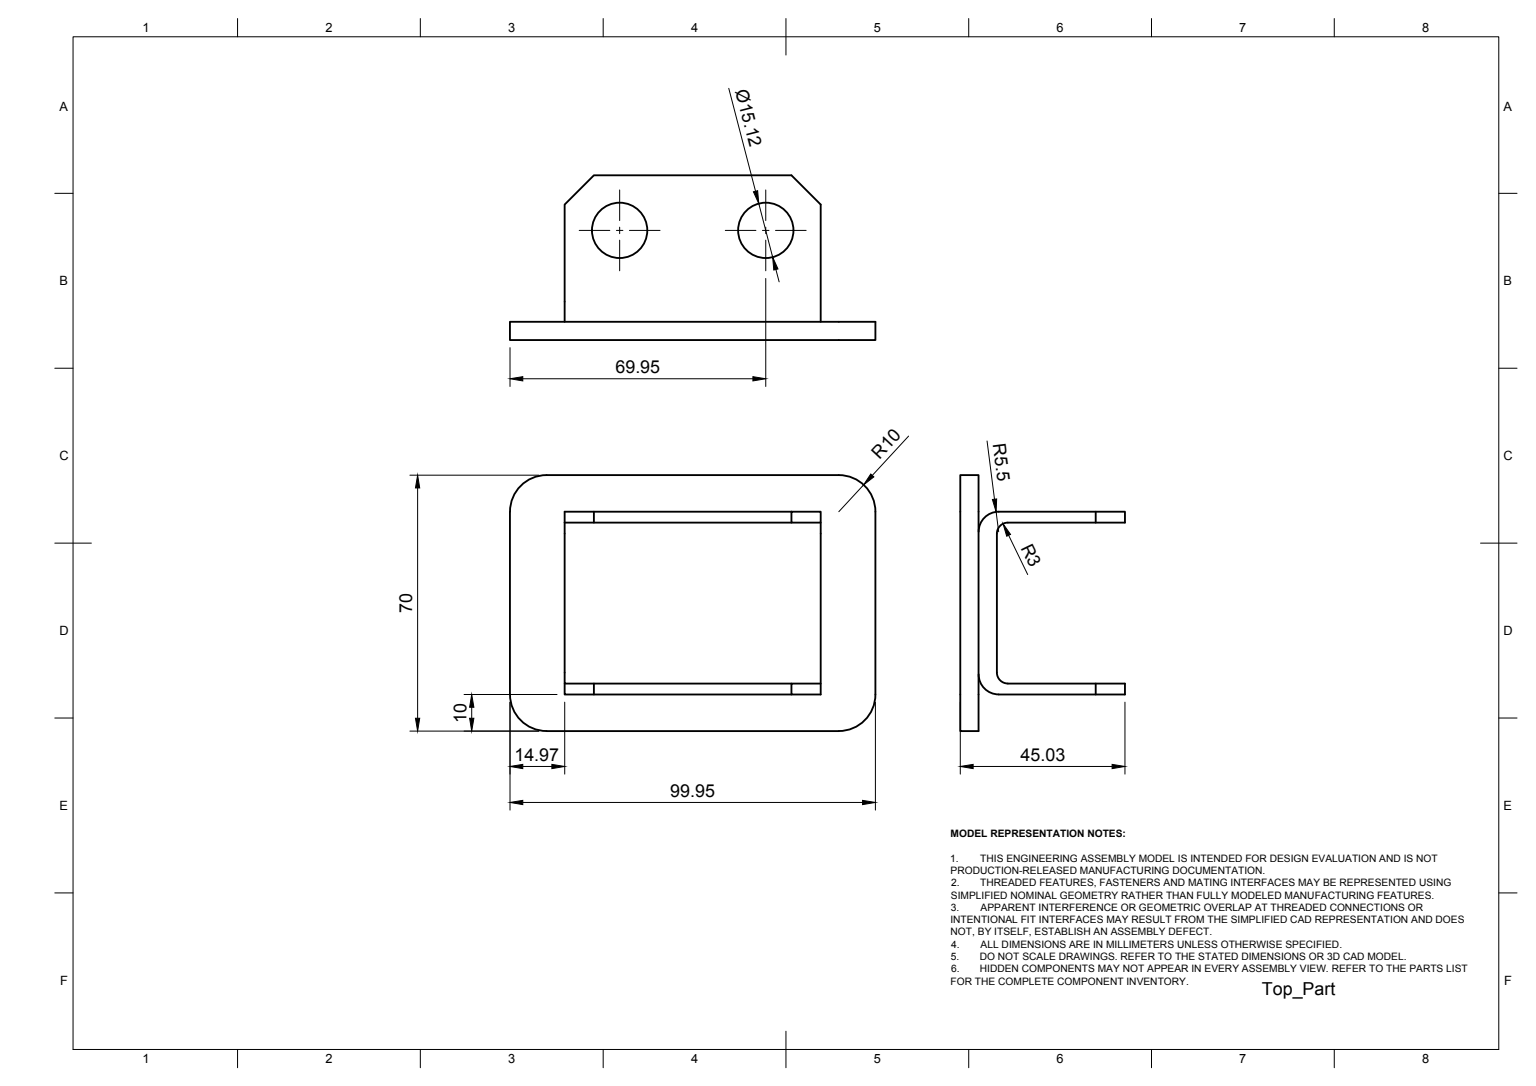
ISO-10303-21;
HEADER;
/* Generated by software containing ST-Developer
 * from STEP Tools, Inc. (www.steptools.com) 
 */

FILE_DESCRIPTION(
/* description */ (''),
/* implementation_level */ '2;1');

FILE_NAME(
/* name */ 'Top_Part.step',
/* time_stamp */ '2026-10-06T13:41:14-07:00',
/* author */ (''),
/* organization */ (''),
/* preprocessor_version */ 'ST-DEVELOPER v20.2',
/* originating_system */ 'Autodesk Translation Framework v15.15.0.0',
/* authorisation */ '');

FILE_SCHEMA (('AUTOMOTIVE_DESIGN { 1 0 10303 214 3 1 1 }'));
ENDSEC;

DATA;
#10=MECHANICAL_DESIGN_GEOMETRIC_PRESENTATION_REPRESENTATION('',(#1966),#279266);
#1948=SHAPE_REPRESENTATION_RELATIONSHIP('SRR','None',#279307,#1957);
#1957=ADVANCED_BREP_SHAPE_REPRESENTATION('',(#1975),#279263);
#1966=STYLED_ITEM('',(#279355),#1975);
#1975=MANIFOLD_SOLID_BREP('Body1',#14944);
#2008=FACE_BOUND('',#3013,.T.);
#2009=FACE_BOUND('',#3014,.T.);
#2010=FACE_BOUND('',#3017,.T.);
#2011=FACE_BOUND('',#3018,.T.);
#2012=FACE_BOUND('',#3030,.T.);
#2013=FACE_BOUND('',#3035,.T.);
#2014=FACE_BOUND('',#3036,.T.);
#2015=FACE_BOUND('',#3039,.T.);
#2016=FACE_BOUND('',#3040,.T.);
#2081=PLANE('',#15559);
#2082=PLANE('',#15563);
#2083=PLANE('',#15567);
#2084=PLANE('',#15572);
#2085=PLANE('',#15575);
#2086=PLANE('',#15576);
#2087=PLANE('',#15580);
#2088=PLANE('',#15581);
#2089=PLANE('',#15587);
#2090=PLANE('',#15591);
#2091=PLANE('',#15592);
#2092=PLANE('',#15593);
#2093=PLANE('',#15594);
#2094=PLANE('',#15597);
#2095=PLANE('',#15601);
#2096=PLANE('',#15603);
#2097=PLANE('',#15605);
#2098=PLANE('',#15606);
#2099=PLANE('',#15607);
#2506=FACE_OUTER_BOUND('',#3006,.T.);
#2507=FACE_OUTER_BOUND('',#3007,.T.);
#2508=FACE_OUTER_BOUND('',#3008,.T.);
#2509=FACE_OUTER_BOUND('',#3009,.T.);
#2510=FACE_OUTER_BOUND('',#3010,.T.);
#2511=FACE_OUTER_BOUND('',#3011,.T.);
#2512=FACE_OUTER_BOUND('',#3012,.T.);
#2513=FACE_OUTER_BOUND('',#3015,.T.);
#2514=FACE_OUTER_BOUND('',#3016,.T.);
#2515=FACE_OUTER_BOUND('',#3019,.T.);
#2516=FACE_OUTER_BOUND('',#3020,.T.);
#2517=FACE_OUTER_BOUND('',#3021,.T.);
#2518=FACE_OUTER_BOUND('',#3022,.T.);
#2519=FACE_OUTER_BOUND('',#3023,.T.);
#2520=FACE_OUTER_BOUND('',#3024,.T.);
#2521=FACE_OUTER_BOUND('',#3025,.T.);
#2522=FACE_OUTER_BOUND('',#3026,.T.);
#2523=FACE_OUTER_BOUND('',#3027,.T.);
#2524=FACE_OUTER_BOUND('',#3028,.T.);
#2525=FACE_OUTER_BOUND('',#3029,.T.);
#2526=FACE_OUTER_BOUND('',#3031,.T.);
#2527=FACE_OUTER_BOUND('',#3032,.T.);
#2528=FACE_OUTER_BOUND('',#3033,.T.);
#2529=FACE_OUTER_BOUND('',#3034,.T.);
#2530=FACE_OUTER_BOUND('',#3037,.T.);
#2531=FACE_OUTER_BOUND('',#3038,.T.);
#2532=FACE_OUTER_BOUND('',#3041,.T.);
#2533=FACE_OUTER_BOUND('',#3042,.T.);
#2534=FACE_OUTER_BOUND('',#3043,.T.);
#2535=FACE_OUTER_BOUND('',#3044,.T.);
#2536=FACE_OUTER_BOUND('',#3045,.T.);
#3006=EDGE_LOOP('',(#13550,#13551,#13552,#13553));
#3007=EDGE_LOOP('',(#13554,#13555,#13556,#13557));
#3008=EDGE_LOOP('',(#13558,#13559,#13560,#13561));
#3009=EDGE_LOOP('',(#13562,#13563,#13564,#13565));
#3010=EDGE_LOOP('',(#13566,#13567,#13568,#13569));
#3011=EDGE_LOOP('',(#13570,#13571,#13572,#13573));
#3012=EDGE_LOOP('',(#13574,#13575,#13576,#13577,#13578,#13579));
#3013=EDGE_LOOP('',(#13580));
#3014=EDGE_LOOP('',(#13581));
#3015=EDGE_LOOP('',(#13582,#13583,#13584,#13585));
#3016=EDGE_LOOP('',(#13586,#13587,#13588,#13589,#13590,#13591));
#3017=EDGE_LOOP('',(#13592));
#3018=EDGE_LOOP('',(#13593));
#3019=EDGE_LOOP('',(#13594,#13595,#13596,#13597));
#3020=EDGE_LOOP('',(#13598,#13599,#13600,#13601));
#3021=EDGE_LOOP('',(#13602,#13603,#13604,#13605));
#3022=EDGE_LOOP('',(#13606,#13607,#13608,#13609));
#3023=EDGE_LOOP('',(#13610,#13611,#13612,#13613));
#3024=EDGE_LOOP('',(#13614,#13615,#13616,#13617,#13618,#13619,#13620,#13621,
#13622,#13623,#13624,#13625));
#3025=EDGE_LOOP('',(#13626,#13627,#13628,#13629));
#3026=EDGE_LOOP('',(#13630,#13631,#13632,#13633));
#3027=EDGE_LOOP('',(#13634,#13635,#13636,#13637));
#3028=EDGE_LOOP('',(#13638,#13639,#13640,#13641));
#3029=EDGE_LOOP('',(#13642,#13643,#13644,#13645,#13646,#13647,#13648,#13649));
#3030=EDGE_LOOP('',(#13650,#13651,#13652,#13653));
#3031=EDGE_LOOP('',(#13654,#13655,#13656,#13657));
#3032=EDGE_LOOP('',(#13658,#13659,#13660,#13661,#13662,#13663,#13664,#13665));
#3033=EDGE_LOOP('',(#13666,#13667,#13668,#13669));
#3034=EDGE_LOOP('',(#13670,#13671,#13672,#13673,#13674,#13675));
#3035=EDGE_LOOP('',(#13676));
#3036=EDGE_LOOP('',(#13677));
#3037=EDGE_LOOP('',(#13678,#13679,#13680,#13681));
#3038=EDGE_LOOP('',(#13682,#13683,#13684,#13685,#13686,#13687));
#3039=EDGE_LOOP('',(#13688));
#3040=EDGE_LOOP('',(#13689));
#3041=EDGE_LOOP('',(#13690,#13691,#13692,#13693,#13694,#13695,#13696,#13697,
#13698,#13699,#13700,#13701));
#3042=EDGE_LOOP('',(#13702,#13703,#13704,#13705));
#3043=EDGE_LOOP('',(#13706,#13707,#13708,#13709));
#3044=EDGE_LOOP('',(#13710,#13711,#13712,#13713));
#3045=EDGE_LOOP('',(#13714,#13715,#13716,#13717));
#3525=LINE('',#240639,#4053);
#3526=LINE('',#240642,#4054);
#3527=LINE('',#240647,#4055);
#3528=LINE('',#240652,#4056);
#3529=LINE('',#240654,#4057);
#3530=LINE('',#240656,#4058);
#3531=LINE('',#240657,#4059);
#3532=LINE('',#240663,#4060);
#3533=LINE('',#240666,#4061);
#3534=LINE('',#240668,#4062);
#3535=LINE('',#240669,#4063);
#3536=LINE('',#240673,#4064);
#3537=LINE('',#240677,#4065);
#3538=LINE('',#240680,#4066);
#3539=LINE('',#240682,#4067);
#3540=LINE('',#240684,#4068);
#3541=LINE('',#240685,#4069);
#3542=LINE('',#240693,#4070);
#3543=LINE('',#240696,#4071);
#3544=LINE('',#240699,#4072);
#3545=LINE('',#240701,#4073);
#3546=LINE('',#240702,#4074);
#3547=LINE('',#240703,#4075);
#3548=LINE('',#240707,#4076);
#3549=LINE('',#240709,#4077);
#3550=LINE('',#240711,#4078);
#3551=LINE('',#240717,#4079);
#3552=LINE('',#240720,#4080);
#3553=LINE('',#240722,#4081);
#3554=LINE('',#240723,#4082);
#3555=LINE('',#240728,#4083);
#3556=LINE('',#240730,#4084);
#3557=LINE('',#240734,#4085);
#3558=LINE('',#240736,#4086);
#3559=LINE('',#240737,#4087);
#3560=LINE('',#240742,#4088);
#3561=LINE('',#240746,#4089);
#3562=LINE('',#240748,#4090);
#3563=LINE('',#240749,#4091);
#3564=LINE('',#240755,#4092);
#3565=LINE('',#240758,#4093);
#3566=LINE('',#240760,#4094);
#3567=LINE('',#240761,#4095);
#3568=LINE('',#240763,#4096);
#3569=LINE('',#240765,#4097);
#3570=LINE('',#240766,#4098);
#3571=LINE('',#240768,#4099);
#3572=LINE('',#240772,#4100);
#3573=LINE('',#240774,#4101);
#3574=LINE('',#240778,#4102);
#3575=LINE('',#240780,#4103);
#3576=LINE('',#240781,#4104);
#3577=LINE('',#240787,#4105);
#3578=LINE('',#240790,#4106);
#3579=LINE('',#240792,#4107);
#3580=LINE('',#240793,#4108);
#3581=LINE('',#240797,#4109);
#3582=LINE('',#240798,#4110);
#3583=LINE('',#240800,#4111);
#3584=LINE('',#240802,#4112);
#4053=VECTOR('',#17119,10.);
#4054=VECTOR('',#17122,10.);
#4055=VECTOR('',#17127,7.55784864301595);
#4056=VECTOR('',#17132,10.);
#4057=VECTOR('',#17133,10.);
#4058=VECTOR('',#17134,9.99999999999999);
#4059=VECTOR('',#17135,10.);
#4060=VECTOR('',#17140,10.);
#4061=VECTOR('',#17143,10.);
#4062=VECTOR('',#17146,10.);
#4063=VECTOR('',#17147,10.);
#4064=VECTOR('',#17150,10.);
#4065=VECTOR('',#17153,10.);
#4066=VECTOR('',#17158,10.);
#4067=VECTOR('',#17159,10.);
#4068=VECTOR('',#17160,10.);
#4069=VECTOR('',#17161,10.);
#4070=VECTOR('',#17168,10.);
#4071=VECTOR('',#17171,10.);
#4072=VECTOR('',#17174,10.);
#4073=VECTOR('',#17175,9.99999999999999);
#4074=VECTOR('',#17176,10.);
#4075=VECTOR('',#17177,10.);
#4076=VECTOR('',#17182,7.55784864301595);
#4077=VECTOR('',#17185,10.);
#4078=VECTOR('',#17188,10.);
#4079=VECTOR('',#17193,10.);
#4080=VECTOR('',#17196,10.);
#4081=VECTOR('',#17199,10.);
#4082=VECTOR('',#17200,10.);
#4083=VECTOR('',#17205,10.);
#4084=VECTOR('',#17206,10.);
#4085=VECTOR('',#17209,10.);
#4086=VECTOR('',#17210,10.);
#4087=VECTOR('',#17211,10.);
#4088=VECTOR('',#17216,7.55784864301595);
#4089=VECTOR('',#17221,10.);
#4090=VECTOR('',#17222,10.);
#4091=VECTOR('',#17223,9.99999999999999);
#4092=VECTOR('',#17228,10.);
#4093=VECTOR('',#17231,10.);
#4094=VECTOR('',#17234,10.);
#4095=VECTOR('',#17235,10.);
#4096=VECTOR('',#17238,10.);
#4097=VECTOR('',#17239,10.);
#4098=VECTOR('',#17240,10.);
#4099=VECTOR('',#17243,10.);
#4100=VECTOR('',#17248,10.);
#4101=VECTOR('',#17249,10.);
#4102=VECTOR('',#17254,10.);
#4103=VECTOR('',#17255,10.);
#4104=VECTOR('',#17256,10.);
#4105=VECTOR('',#17263,10.);
#4106=VECTOR('',#17266,10.);
#4107=VECTOR('',#17267,9.99999999999999);
#4108=VECTOR('',#17268,10.);
#4109=VECTOR('',#17273,10.);
#4110=VECTOR('',#17274,10.);
#4111=VECTOR('',#17277,7.55784864301595);
#4112=VECTOR('',#17280,10.);
#4260=CIRCLE('',#15554,10.);
#4261=CIRCLE('',#15555,10.);
#4262=CIRCLE('',#15557,7.55784864301595);
#4263=CIRCLE('',#15558,7.55784864301595);
#4264=CIRCLE('',#15561,10.);
#4265=CIRCLE('',#15562,10.);
#4266=CIRCLE('',#15565,3.);
#4267=CIRCLE('',#15566,3.);
#4268=CIRCLE('',#15568,7.55784864301595);
#4269=CIRCLE('',#15570,5.5);
#4270=CIRCLE('',#15571,5.5);
#4271=CIRCLE('',#15573,7.55784864301595);
#4272=CIRCLE('',#15578,10.);
#4273=CIRCLE('',#15579,10.);
#4274=CIRCLE('',#15582,5.5);
#4275=CIRCLE('',#15583,3.);
#4276=CIRCLE('',#15585,7.55784864301595);
#4277=CIRCLE('',#15586,7.55784864301595);
#4278=CIRCLE('',#15589,10.);
#4279=CIRCLE('',#15590,10.);
#4280=CIRCLE('',#15596,3.);
#4281=CIRCLE('',#15598,7.55784864301595);
#4282=CIRCLE('',#15600,5.5);
#4283=CIRCLE('',#15602,7.55784864301595);
#6207=VERTEX_POINT('',#240635);
#6208=VERTEX_POINT('',#240636);
#6209=VERTEX_POINT('',#240638);
#6210=VERTEX_POINT('',#240640);
#6211=VERTEX_POINT('',#240644);
#6212=VERTEX_POINT('',#240646);
#6213=VERTEX_POINT('',#240650);
#6214=VERTEX_POINT('',#240651);
#6215=VERTEX_POINT('',#240653);
#6216=VERTEX_POINT('',#240655);
#6217=VERTEX_POINT('',#240659);
#6218=VERTEX_POINT('',#240660);
#6219=VERTEX_POINT('',#240662);
#6220=VERTEX_POINT('',#240664);
#6221=VERTEX_POINT('',#240671);
#6222=VERTEX_POINT('',#240672);
#6223=VERTEX_POINT('',#240674);
#6224=VERTEX_POINT('',#240676);
#6225=VERTEX_POINT('',#240681);
#6226=VERTEX_POINT('',#240683);
#6227=VERTEX_POINT('',#240686);
#6228=VERTEX_POINT('',#240689);
#6229=VERTEX_POINT('',#240690);
#6230=VERTEX_POINT('',#240692);
#6231=VERTEX_POINT('',#240694);
#6232=VERTEX_POINT('',#240698);
#6233=VERTEX_POINT('',#240700);
#6234=VERTEX_POINT('',#240704);
#6235=VERTEX_POINT('',#240713);
#6236=VERTEX_POINT('',#240714);
#6237=VERTEX_POINT('',#240716);
#6238=VERTEX_POINT('',#240718);
#6239=VERTEX_POINT('',#240725);
#6240=VERTEX_POINT('',#240726);
#6241=VERTEX_POINT('',#240729);
#6242=VERTEX_POINT('',#240731);
#6243=VERTEX_POINT('',#240733);
#6244=VERTEX_POINT('',#240735);
#6245=VERTEX_POINT('',#240739);
#6246=VERTEX_POINT('',#240741);
#6247=VERTEX_POINT('',#240745);
#6248=VERTEX_POINT('',#240747);
#6249=VERTEX_POINT('',#240751);
#6250=VERTEX_POINT('',#240752);
#6251=VERTEX_POINT('',#240754);
#6252=VERTEX_POINT('',#240756);
#6253=VERTEX_POINT('',#240764);
#6254=VERTEX_POINT('',#240771);
#6255=VERTEX_POINT('',#240773);
#6256=VERTEX_POINT('',#240777);
#6257=VERTEX_POINT('',#240779);
#6258=VERTEX_POINT('',#240782);
#6259=VERTEX_POINT('',#240785);
#6260=VERTEX_POINT('',#240789);
#6261=VERTEX_POINT('',#240791);
#6262=VERTEX_POINT('',#240794);
#8700=EDGE_CURVE('',#6207,#6208,#4260,.T.);
#8701=EDGE_CURVE('',#6209,#6207,#3525,.T.);
#8702=EDGE_CURVE('',#6210,#6209,#4261,.T.);
#8703=EDGE_CURVE('',#6208,#6210,#3526,.T.);
#8704=EDGE_CURVE('',#6211,#6211,#4262,.T.);
#8705=EDGE_CURVE('',#6211,#6212,#3527,.T.);
#8706=EDGE_CURVE('',#6212,#6212,#4263,.T.);
#8707=EDGE_CURVE('',#6213,#6214,#3528,.T.);
#8708=EDGE_CURVE('',#6213,#6215,#3529,.T.);
#8709=EDGE_CURVE('',#6215,#6216,#3530,.T.);
#8710=EDGE_CURVE('',#6214,#6216,#3531,.T.);
#8711=EDGE_CURVE('',#6217,#6218,#4264,.T.);
#8712=EDGE_CURVE('',#6218,#6219,#3532,.T.);
#8713=EDGE_CURVE('',#6219,#6220,#4265,.T.);
#8714=EDGE_CURVE('',#6220,#6217,#3533,.T.);
#8715=EDGE_CURVE('',#6218,#6208,#3534,.T.);
#8716=EDGE_CURVE('',#6219,#6210,#3535,.T.);
#8717=EDGE_CURVE('',#6221,#6222,#3536,.T.);
#8718=EDGE_CURVE('',#6222,#6223,#4266,.T.);
#8719=EDGE_CURVE('',#6223,#6224,#3537,.T.);
#8720=EDGE_CURVE('',#6221,#6224,#4267,.T.);
#8721=EDGE_CURVE('',#6221,#6213,#3538,.T.);
#8722=EDGE_CURVE('',#6214,#6225,#3539,.T.);
#8723=EDGE_CURVE('',#6226,#6225,#3540,.T.);
#8724=EDGE_CURVE('',#6222,#6226,#3541,.T.);
#8725=EDGE_CURVE('',#6227,#6227,#4268,.T.);
#8726=EDGE_CURVE('',#6228,#6229,#4269,.T.);
#8727=EDGE_CURVE('',#6229,#6230,#3542,.T.);
#8728=EDGE_CURVE('',#6231,#6230,#4270,.T.);
#8729=EDGE_CURVE('',#6231,#6228,#3543,.T.);
#8730=EDGE_CURVE('',#6229,#6232,#3544,.T.);
#8731=EDGE_CURVE('',#6232,#6233,#3545,.T.);
#8732=EDGE_CURVE('',#6233,#6216,#3546,.T.);
#8733=EDGE_CURVE('',#6230,#6215,#3547,.T.);
#8734=EDGE_CURVE('',#6234,#6234,#4271,.T.);
#8735=EDGE_CURVE('',#6227,#6234,#3548,.T.);
#8736=EDGE_CURVE('',#6225,#6233,#3549,.T.);
#8737=EDGE_CURVE('',#6226,#6232,#3550,.T.);
#8738=EDGE_CURVE('',#6235,#6236,#4272,.T.);
#8739=EDGE_CURVE('',#6236,#6237,#3551,.T.);
#8740=EDGE_CURVE('',#6237,#6238,#4273,.T.);
#8741=EDGE_CURVE('',#6238,#6235,#3552,.T.);
#8742=EDGE_CURVE('',#6209,#6238,#3553,.T.);
#8743=EDGE_CURVE('',#6207,#6235,#3554,.T.);
#8744=EDGE_CURVE('',#6239,#6240,#4274,.T.);
#8745=EDGE_CURVE('',#6231,#6239,#3555,.T.);
#8746=EDGE_CURVE('',#6241,#6224,#3556,.T.);
#8747=EDGE_CURVE('',#6242,#6241,#4275,.T.);
#8748=EDGE_CURVE('',#6242,#6243,#3557,.T.);
#8749=EDGE_CURVE('',#6243,#6244,#3558,.T.);
#8750=EDGE_CURVE('',#6240,#6244,#3559,.T.);
#8751=EDGE_CURVE('',#6245,#6245,#4276,.T.);
#8752=EDGE_CURVE('',#6245,#6246,#3560,.T.);
#8753=EDGE_CURVE('',#6246,#6246,#4277,.T.);
#8754=EDGE_CURVE('',#6243,#6247,#3561,.T.);
#8755=EDGE_CURVE('',#6247,#6248,#3562,.T.);
#8756=EDGE_CURVE('',#6244,#6248,#3563,.T.);
#8757=EDGE_CURVE('',#6249,#6250,#4278,.T.);
#8758=EDGE_CURVE('',#6251,#6249,#3564,.T.);
#8759=EDGE_CURVE('',#6252,#6251,#4279,.T.);
#8760=EDGE_CURVE('',#6250,#6252,#3565,.T.);
#8761=EDGE_CURVE('',#6252,#6237,#3566,.T.);
#8762=EDGE_CURVE('',#6250,#6236,#3567,.T.);
#8763=EDGE_CURVE('',#6249,#6217,#3568,.T.);
#8764=EDGE_CURVE('',#6239,#6253,#3569,.T.);
#8765=EDGE_CURVE('',#6253,#6228,#3570,.T.);
#8766=EDGE_CURVE('',#6251,#6220,#3571,.T.);
#8767=EDGE_CURVE('',#6242,#6254,#3572,.T.);
#8768=EDGE_CURVE('',#6255,#6241,#3573,.T.);
#8769=EDGE_CURVE('',#6254,#6255,#4280,.T.);
#8770=EDGE_CURVE('',#6254,#6256,#3574,.T.);
#8771=EDGE_CURVE('',#6256,#6257,#3575,.T.);
#8772=EDGE_CURVE('',#6247,#6257,#3576,.T.);
#8773=EDGE_CURVE('',#6258,#6258,#4281,.T.);
#8774=EDGE_CURVE('',#6253,#6259,#4282,.T.);
#8775=EDGE_CURVE('',#6259,#6240,#3577,.T.);
#8776=EDGE_CURVE('',#6260,#6248,#3578,.T.);
#8777=EDGE_CURVE('',#6261,#6260,#3579,.T.);
#8778=EDGE_CURVE('',#6259,#6261,#3580,.T.);
#8779=EDGE_CURVE('',#6262,#6262,#4283,.T.);
#8780=EDGE_CURVE('',#6256,#6261,#3581,.T.);
#8781=EDGE_CURVE('',#6255,#6223,#3582,.T.);
#8782=EDGE_CURVE('',#6262,#6258,#3583,.T.);
#8783=EDGE_CURVE('',#6257,#6260,#3584,.T.);
#13550=ORIENTED_EDGE('',*,*,#8700,.F.);
#13551=ORIENTED_EDGE('',*,*,#8701,.F.);
#13552=ORIENTED_EDGE('',*,*,#8702,.F.);
#13553=ORIENTED_EDGE('',*,*,#8703,.F.);
#13554=ORIENTED_EDGE('',*,*,#8704,.T.);
#13555=ORIENTED_EDGE('',*,*,#8705,.T.);
#13556=ORIENTED_EDGE('',*,*,#8706,.F.);
#13557=ORIENTED_EDGE('',*,*,#8705,.F.);
#13558=ORIENTED_EDGE('',*,*,#8707,.F.);
#13559=ORIENTED_EDGE('',*,*,#8708,.T.);
#13560=ORIENTED_EDGE('',*,*,#8709,.T.);
#13561=ORIENTED_EDGE('',*,*,#8710,.F.);
#13562=ORIENTED_EDGE('',*,*,#8711,.T.);
#13563=ORIENTED_EDGE('',*,*,#8712,.T.);
#13564=ORIENTED_EDGE('',*,*,#8713,.T.);
#13565=ORIENTED_EDGE('',*,*,#8714,.T.);
#13566=ORIENTED_EDGE('',*,*,#8712,.F.);
#13567=ORIENTED_EDGE('',*,*,#8715,.T.);
#13568=ORIENTED_EDGE('',*,*,#8703,.T.);
#13569=ORIENTED_EDGE('',*,*,#8716,.F.);
#13570=ORIENTED_EDGE('',*,*,#8717,.T.);
#13571=ORIENTED_EDGE('',*,*,#8718,.T.);
#13572=ORIENTED_EDGE('',*,*,#8719,.T.);
#13573=ORIENTED_EDGE('',*,*,#8720,.F.);
#13574=ORIENTED_EDGE('',*,*,#8717,.F.);
#13575=ORIENTED_EDGE('',*,*,#8721,.T.);
#13576=ORIENTED_EDGE('',*,*,#8707,.T.);
#13577=ORIENTED_EDGE('',*,*,#8722,.T.);
#13578=ORIENTED_EDGE('',*,*,#8723,.F.);
#13579=ORIENTED_EDGE('',*,*,#8724,.F.);
#13580=ORIENTED_EDGE('',*,*,#8706,.T.);
#13581=ORIENTED_EDGE('',*,*,#8725,.F.);
#13582=ORIENTED_EDGE('',*,*,#8726,.T.);
#13583=ORIENTED_EDGE('',*,*,#8727,.T.);
#13584=ORIENTED_EDGE('',*,*,#8728,.F.);
#13585=ORIENTED_EDGE('',*,*,#8729,.T.);
#13586=ORIENTED_EDGE('',*,*,#8727,.F.);
#13587=ORIENTED_EDGE('',*,*,#8730,.T.);
#13588=ORIENTED_EDGE('',*,*,#8731,.T.);
#13589=ORIENTED_EDGE('',*,*,#8732,.T.);
#13590=ORIENTED_EDGE('',*,*,#8709,.F.);
#13591=ORIENTED_EDGE('',*,*,#8733,.F.);
#13592=ORIENTED_EDGE('',*,*,#8704,.F.);
#13593=ORIENTED_EDGE('',*,*,#8734,.T.);
#13594=ORIENTED_EDGE('',*,*,#8725,.T.);
#13595=ORIENTED_EDGE('',*,*,#8735,.T.);
#13596=ORIENTED_EDGE('',*,*,#8734,.F.);
#13597=ORIENTED_EDGE('',*,*,#8735,.F.);
#13598=ORIENTED_EDGE('',*,*,#8722,.F.);
#13599=ORIENTED_EDGE('',*,*,#8710,.T.);
#13600=ORIENTED_EDGE('',*,*,#8732,.F.);
#13601=ORIENTED_EDGE('',*,*,#8736,.F.);
#13602=ORIENTED_EDGE('',*,*,#8723,.T.);
#13603=ORIENTED_EDGE('',*,*,#8736,.T.);
#13604=ORIENTED_EDGE('',*,*,#8731,.F.);
#13605=ORIENTED_EDGE('',*,*,#8737,.F.);
#13606=ORIENTED_EDGE('',*,*,#8738,.T.);
#13607=ORIENTED_EDGE('',*,*,#8739,.T.);
#13608=ORIENTED_EDGE('',*,*,#8740,.T.);
#13609=ORIENTED_EDGE('',*,*,#8741,.T.);
#13610=ORIENTED_EDGE('',*,*,#8741,.F.);
#13611=ORIENTED_EDGE('',*,*,#8742,.F.);
#13612=ORIENTED_EDGE('',*,*,#8701,.T.);
#13613=ORIENTED_EDGE('',*,*,#8743,.T.);
#13614=ORIENTED_EDGE('',*,*,#8744,.F.);
#13615=ORIENTED_EDGE('',*,*,#8745,.F.);
#13616=ORIENTED_EDGE('',*,*,#8728,.T.);
#13617=ORIENTED_EDGE('',*,*,#8733,.T.);
#13618=ORIENTED_EDGE('',*,*,#8708,.F.);
#13619=ORIENTED_EDGE('',*,*,#8721,.F.);
#13620=ORIENTED_EDGE('',*,*,#8720,.T.);
#13621=ORIENTED_EDGE('',*,*,#8746,.F.);
#13622=ORIENTED_EDGE('',*,*,#8747,.F.);
#13623=ORIENTED_EDGE('',*,*,#8748,.T.);
#13624=ORIENTED_EDGE('',*,*,#8749,.T.);
#13625=ORIENTED_EDGE('',*,*,#8750,.F.);
#13626=ORIENTED_EDGE('',*,*,#8751,.T.);
#13627=ORIENTED_EDGE('',*,*,#8752,.T.);
#13628=ORIENTED_EDGE('',*,*,#8753,.F.);
#13629=ORIENTED_EDGE('',*,*,#8752,.F.);
#13630=ORIENTED_EDGE('',*,*,#8754,.T.);
#13631=ORIENTED_EDGE('',*,*,#8755,.T.);
#13632=ORIENTED_EDGE('',*,*,#8756,.F.);
#13633=ORIENTED_EDGE('',*,*,#8749,.F.);
#13634=ORIENTED_EDGE('',*,*,#8757,.F.);
#13635=ORIENTED_EDGE('',*,*,#8758,.F.);
#13636=ORIENTED_EDGE('',*,*,#8759,.F.);
#13637=ORIENTED_EDGE('',*,*,#8760,.F.);
#13638=ORIENTED_EDGE('',*,*,#8760,.T.);
#13639=ORIENTED_EDGE('',*,*,#8761,.T.);
#13640=ORIENTED_EDGE('',*,*,#8739,.F.);
#13641=ORIENTED_EDGE('',*,*,#8762,.F.);
#13642=ORIENTED_EDGE('',*,*,#8743,.F.);
#13643=ORIENTED_EDGE('',*,*,#8700,.T.);
#13644=ORIENTED_EDGE('',*,*,#8715,.F.);
#13645=ORIENTED_EDGE('',*,*,#8711,.F.);
#13646=ORIENTED_EDGE('',*,*,#8763,.F.);
#13647=ORIENTED_EDGE('',*,*,#8757,.T.);
#13648=ORIENTED_EDGE('',*,*,#8762,.T.);
#13649=ORIENTED_EDGE('',*,*,#8738,.F.);
#13650=ORIENTED_EDGE('',*,*,#8745,.T.);
#13651=ORIENTED_EDGE('',*,*,#8764,.T.);
#13652=ORIENTED_EDGE('',*,*,#8765,.T.);
#13653=ORIENTED_EDGE('',*,*,#8729,.F.);
#13654=ORIENTED_EDGE('',*,*,#8758,.T.);
#13655=ORIENTED_EDGE('',*,*,#8763,.T.);
#13656=ORIENTED_EDGE('',*,*,#8714,.F.);
#13657=ORIENTED_EDGE('',*,*,#8766,.F.);
#13658=ORIENTED_EDGE('',*,*,#8759,.T.);
#13659=ORIENTED_EDGE('',*,*,#8766,.T.);
#13660=ORIENTED_EDGE('',*,*,#8713,.F.);
#13661=ORIENTED_EDGE('',*,*,#8716,.T.);
#13662=ORIENTED_EDGE('',*,*,#8702,.T.);
#13663=ORIENTED_EDGE('',*,*,#8742,.T.);
#13664=ORIENTED_EDGE('',*,*,#8740,.F.);
#13665=ORIENTED_EDGE('',*,*,#8761,.F.);
#13666=ORIENTED_EDGE('',*,*,#8767,.F.);
#13667=ORIENTED_EDGE('',*,*,#8747,.T.);
#13668=ORIENTED_EDGE('',*,*,#8768,.F.);
#13669=ORIENTED_EDGE('',*,*,#8769,.F.);
#13670=ORIENTED_EDGE('',*,*,#8767,.T.);
#13671=ORIENTED_EDGE('',*,*,#8770,.T.);
#13672=ORIENTED_EDGE('',*,*,#8771,.T.);
#13673=ORIENTED_EDGE('',*,*,#8772,.F.);
#13674=ORIENTED_EDGE('',*,*,#8754,.F.);
#13675=ORIENTED_EDGE('',*,*,#8748,.F.);
#13676=ORIENTED_EDGE('',*,*,#8751,.F.);
#13677=ORIENTED_EDGE('',*,*,#8773,.T.);
#13678=ORIENTED_EDGE('',*,*,#8774,.F.);
#13679=ORIENTED_EDGE('',*,*,#8764,.F.);
#13680=ORIENTED_EDGE('',*,*,#8744,.T.);
#13681=ORIENTED_EDGE('',*,*,#8775,.F.);
#13682=ORIENTED_EDGE('',*,*,#8775,.T.);
#13683=ORIENTED_EDGE('',*,*,#8750,.T.);
#13684=ORIENTED_EDGE('',*,*,#8756,.T.);
#13685=ORIENTED_EDGE('',*,*,#8776,.F.);
#13686=ORIENTED_EDGE('',*,*,#8777,.F.);
#13687=ORIENTED_EDGE('',*,*,#8778,.F.);
#13688=ORIENTED_EDGE('',*,*,#8753,.T.);
#13689=ORIENTED_EDGE('',*,*,#8779,.F.);
#13690=ORIENTED_EDGE('',*,*,#8774,.T.);
#13691=ORIENTED_EDGE('',*,*,#8778,.T.);
#13692=ORIENTED_EDGE('',*,*,#8780,.F.);
#13693=ORIENTED_EDGE('',*,*,#8770,.F.);
#13694=ORIENTED_EDGE('',*,*,#8769,.T.);
#13695=ORIENTED_EDGE('',*,*,#8781,.T.);
#13696=ORIENTED_EDGE('',*,*,#8718,.F.);
#13697=ORIENTED_EDGE('',*,*,#8724,.T.);
#13698=ORIENTED_EDGE('',*,*,#8737,.T.);
#13699=ORIENTED_EDGE('',*,*,#8730,.F.);
#13700=ORIENTED_EDGE('',*,*,#8726,.F.);
#13701=ORIENTED_EDGE('',*,*,#8765,.F.);
#13702=ORIENTED_EDGE('',*,*,#8779,.T.);
#13703=ORIENTED_EDGE('',*,*,#8782,.T.);
#13704=ORIENTED_EDGE('',*,*,#8773,.F.);
#13705=ORIENTED_EDGE('',*,*,#8782,.F.);
#13706=ORIENTED_EDGE('',*,*,#8772,.T.);
#13707=ORIENTED_EDGE('',*,*,#8783,.T.);
#13708=ORIENTED_EDGE('',*,*,#8776,.T.);
#13709=ORIENTED_EDGE('',*,*,#8755,.F.);
#13710=ORIENTED_EDGE('',*,*,#8771,.F.);
#13711=ORIENTED_EDGE('',*,*,#8780,.T.);
#13712=ORIENTED_EDGE('',*,*,#8777,.T.);
#13713=ORIENTED_EDGE('',*,*,#8783,.F.);
#13714=ORIENTED_EDGE('',*,*,#8768,.T.);
#13715=ORIENTED_EDGE('',*,*,#8746,.T.);
#13716=ORIENTED_EDGE('',*,*,#8719,.F.);
#13717=ORIENTED_EDGE('',*,*,#8781,.F.);
#14427=CYLINDRICAL_SURFACE('',#15553,10.);
#14428=CYLINDRICAL_SURFACE('',#15556,7.55784864301595);
#14429=CYLINDRICAL_SURFACE('',#15560,10.);
#14430=CYLINDRICAL_SURFACE('',#15564,3.);
#14431=CYLINDRICAL_SURFACE('',#15569,5.5);
#14432=CYLINDRICAL_SURFACE('',#15574,7.55784864301595);
#14433=CYLINDRICAL_SURFACE('',#15577,10.);
#14434=CYLINDRICAL_SURFACE('',#15584,7.55784864301595);
#14435=CYLINDRICAL_SURFACE('',#15588,10.);
#14436=CYLINDRICAL_SURFACE('',#15595,3.);
#14437=CYLINDRICAL_SURFACE('',#15599,5.5);
#14438=CYLINDRICAL_SURFACE('',#15604,7.55784864301595);
#14864=ADVANCED_FACE('',(#2506),#14427,.T.);
#14865=ADVANCED_FACE('',(#2507),#14428,.F.);
#14866=ADVANCED_FACE('',(#2508),#2081,.F.);
#14867=ADVANCED_FACE('',(#2509),#14429,.T.);
#14868=ADVANCED_FACE('',(#2510),#2082,.T.);
#14869=ADVANCED_FACE('',(#2511),#14430,.F.);
#14870=ADVANCED_FACE('',(#2512,#2008,#2009),#2083,.T.);
#14871=ADVANCED_FACE('',(#2513),#14431,.T.);
#14872=ADVANCED_FACE('',(#2514,#2010,#2011),#2084,.T.);
#14873=ADVANCED_FACE('',(#2515),#14432,.F.);
#14874=ADVANCED_FACE('',(#2516),#2085,.T.);
#14875=ADVANCED_FACE('',(#2517),#2086,.T.);
#14876=ADVANCED_FACE('',(#2518),#14433,.T.);
#14877=ADVANCED_FACE('',(#2519),#2087,.T.);
#14878=ADVANCED_FACE('',(#2520),#2088,.T.);
#14879=ADVANCED_FACE('',(#2521),#14434,.F.);
#14880=ADVANCED_FACE('',(#2522),#2089,.T.);
#14881=ADVANCED_FACE('',(#2523),#14435,.T.);
#14882=ADVANCED_FACE('',(#2524),#2090,.F.);
#14883=ADVANCED_FACE('',(#2525,#2012),#2091,.F.);
#14884=ADVANCED_FACE('',(#2526),#2092,.F.);
#14885=ADVANCED_FACE('',(#2527),#2093,.F.);
#14886=ADVANCED_FACE('',(#2528),#14436,.F.);
#14887=ADVANCED_FACE('',(#2529,#2013,#2014),#2094,.F.);
#14888=ADVANCED_FACE('',(#2530),#14437,.T.);
#14889=ADVANCED_FACE('',(#2531,#2015,#2016),#2095,.F.);
#14890=ADVANCED_FACE('',(#2532),#2096,.F.);
#14891=ADVANCED_FACE('',(#2533),#14438,.F.);
#14892=ADVANCED_FACE('',(#2534),#2097,.F.);
#14893=ADVANCED_FACE('',(#2535),#2098,.F.);
#14894=ADVANCED_FACE('',(#2536),#2099,.F.);
#14944=CLOSED_SHELL('',(#14864,#14865,#14866,#14867,#14868,#14869,#14870,
#14871,#14872,#14873,#14874,#14875,#14876,#14877,#14878,#14879,#14880,#14881,
#14882,#14883,#14884,#14885,#14886,#14887,#14888,#14889,#14890,#14891,#14892,
#14893,#14894));
#15552=AXIS2_PLACEMENT_3D('',#240633,#17113,#17114);
#15553=AXIS2_PLACEMENT_3D('',#240634,#17115,#17116);
#15554=AXIS2_PLACEMENT_3D('',#240637,#17117,#17118);
#15555=AXIS2_PLACEMENT_3D('',#240641,#17120,#17121);
#15556=AXIS2_PLACEMENT_3D('',#240643,#17123,#17124);
#15557=AXIS2_PLACEMENT_3D('',#240645,#17125,#17126);
#15558=AXIS2_PLACEMENT_3D('',#240648,#17128,#17129);
#15559=AXIS2_PLACEMENT_3D('',#240649,#17130,#17131);
#15560=AXIS2_PLACEMENT_3D('',#240658,#17136,#17137);
#15561=AXIS2_PLACEMENT_3D('',#240661,#17138,#17139);
#15562=AXIS2_PLACEMENT_3D('',#240665,#17141,#17142);
#15563=AXIS2_PLACEMENT_3D('',#240667,#17144,#17145);
#15564=AXIS2_PLACEMENT_3D('',#240670,#17148,#17149);
#15565=AXIS2_PLACEMENT_3D('',#240675,#17151,#17152);
#15566=AXIS2_PLACEMENT_3D('',#240678,#17154,#17155);
#15567=AXIS2_PLACEMENT_3D('',#240679,#17156,#17157);
#15568=AXIS2_PLACEMENT_3D('',#240687,#17162,#17163);
#15569=AXIS2_PLACEMENT_3D('',#240688,#17164,#17165);
#15570=AXIS2_PLACEMENT_3D('',#240691,#17166,#17167);
#15571=AXIS2_PLACEMENT_3D('',#240695,#17169,#17170);
#15572=AXIS2_PLACEMENT_3D('',#240697,#17172,#17173);
#15573=AXIS2_PLACEMENT_3D('',#240705,#17178,#17179);
#15574=AXIS2_PLACEMENT_3D('',#240706,#17180,#17181);
#15575=AXIS2_PLACEMENT_3D('',#240708,#17183,#17184);
#15576=AXIS2_PLACEMENT_3D('',#240710,#17186,#17187);
#15577=AXIS2_PLACEMENT_3D('',#240712,#17189,#17190);
#15578=AXIS2_PLACEMENT_3D('',#240715,#17191,#17192);
#15579=AXIS2_PLACEMENT_3D('',#240719,#17194,#17195);
#15580=AXIS2_PLACEMENT_3D('',#240721,#17197,#17198);
#15581=AXIS2_PLACEMENT_3D('',#240724,#17201,#17202);
#15582=AXIS2_PLACEMENT_3D('',#240727,#17203,#17204);
#15583=AXIS2_PLACEMENT_3D('',#240732,#17207,#17208);
#15584=AXIS2_PLACEMENT_3D('',#240738,#17212,#17213);
#15585=AXIS2_PLACEMENT_3D('',#240740,#17214,#17215);
#15586=AXIS2_PLACEMENT_3D('',#240743,#17217,#17218);
#15587=AXIS2_PLACEMENT_3D('',#240744,#17219,#17220);
#15588=AXIS2_PLACEMENT_3D('',#240750,#17224,#17225);
#15589=AXIS2_PLACEMENT_3D('',#240753,#17226,#17227);
#15590=AXIS2_PLACEMENT_3D('',#240757,#17229,#17230);
#15591=AXIS2_PLACEMENT_3D('',#240759,#17232,#17233);
#15592=AXIS2_PLACEMENT_3D('',#240762,#17236,#17237);
#15593=AXIS2_PLACEMENT_3D('',#240767,#17241,#17242);
#15594=AXIS2_PLACEMENT_3D('',#240769,#17244,#17245);
#15595=AXIS2_PLACEMENT_3D('',#240770,#17246,#17247);
#15596=AXIS2_PLACEMENT_3D('',#240775,#17250,#17251);
#15597=AXIS2_PLACEMENT_3D('',#240776,#17252,#17253);
#15598=AXIS2_PLACEMENT_3D('',#240783,#17257,#17258);
#15599=AXIS2_PLACEMENT_3D('',#240784,#17259,#17260);
#15600=AXIS2_PLACEMENT_3D('',#240786,#17261,#17262);
#15601=AXIS2_PLACEMENT_3D('',#240788,#17264,#17265);
#15602=AXIS2_PLACEMENT_3D('',#240795,#17269,#17270);
#15603=AXIS2_PLACEMENT_3D('',#240796,#17271,#17272);
#15604=AXIS2_PLACEMENT_3D('',#240799,#17275,#17276);
#15605=AXIS2_PLACEMENT_3D('',#240801,#17278,#17279);
#15606=AXIS2_PLACEMENT_3D('',#240803,#17281,#17282);
#15607=AXIS2_PLACEMENT_3D('',#240804,#17283,#17284);
#17113=DIRECTION('axis',(0.,0.,1.));
#17114=DIRECTION('refdir',(1.,0.,0.));
#17115=DIRECTION('center_axis',(0.,0.,1.));
#17116=DIRECTION('ref_axis',(-0.707106781186548,0.707106781186548,0.));
#17117=DIRECTION('center_axis',(0.,0.,-1.));
#17118=DIRECTION('ref_axis',(-0.707106781186548,0.707106781186548,0.));
#17119=DIRECTION('',(0.,0.,-1.));
#17120=DIRECTION('center_axis',(0.,0.,1.));
#17121=DIRECTION('ref_axis',(-0.707106781186548,0.707106781186548,0.));
#17122=DIRECTION('',(0.,0.,1.));
#17123=DIRECTION('center_axis',(0.,-1.,0.));
#17124=DIRECTION('ref_axis',(-1.,0.,0.));
#17125=DIRECTION('center_axis',(0.,1.,0.));
#17126=DIRECTION('ref_axis',(-1.,0.,0.));
#17127=DIRECTION('',(0.,-1.,0.));
#17128=DIRECTION('center_axis',(0.,1.,0.));
#17129=DIRECTION('ref_axis',(-1.,0.,0.));
#17130=DIRECTION('center_axis',(0.707106781186548,0.,0.707106781186548));
#17131=DIRECTION('ref_axis',(0.707106781186548,0.,-0.707106781186548));
#17132=DIRECTION('',(0.707106781186547,0.,-0.707106781186547));
#17133=DIRECTION('',(0.,1.,0.));
#17134=DIRECTION('',(0.707106781186547,0.,-0.707106781186547));
#17135=DIRECTION('',(0.,1.,0.));
#17136=DIRECTION('center_axis',(0.,0.,-1.));
#17137=DIRECTION('ref_axis',(0.707106781186548,0.707106781186548,0.));
#17138=DIRECTION('center_axis',(0.,0.,1.));
#17139=DIRECTION('ref_axis',(0.707106781186548,0.707106781186548,0.));
#17140=DIRECTION('',(0.,0.,1.));
#17141=DIRECTION('center_axis',(0.,0.,-1.));
#17142=DIRECTION('ref_axis',(0.707106781186548,0.707106781186548,0.));
#17143=DIRECTION('',(0.,0.,-1.));
#17144=DIRECTION('center_axis',(0.,1.,0.));
#17145=DIRECTION('ref_axis',(0.,0.,1.));
#17146=DIRECTION('',(-1.,0.,0.));
#17147=DIRECTION('',(-1.,0.,0.));
#17148=DIRECTION('center_axis',(1.,0.,0.));
#17149=DIRECTION('ref_axis',(0.,0.707106781186548,0.707106781186547));
#17150=DIRECTION('',(1.,0.,0.));
#17151=DIRECTION('center_axis',(1.,0.,0.));
#17152=DIRECTION('ref_axis',(0.,0.707106781186548,0.707106781186547));
#17153=DIRECTION('',(-1.,0.,0.));
#17154=DIRECTION('center_axis',(1.,0.,0.));
#17155=DIRECTION('ref_axis',(0.,0.707106781186548,0.707106781186547));
#17156=DIRECTION('center_axis',(0.,-1.,0.));
#17157=DIRECTION('ref_axis',(1.,0.,0.));
#17158=DIRECTION('',(0.,0.,-1.));
#17159=DIRECTION('',(1.,0.,0.));
#17160=DIRECTION('',(-0.707106781186547,0.,-0.707106781186547));
#17161=DIRECTION('',(0.,0.,-1.));
#17162=DIRECTION('center_axis',(0.,-1.,0.));
#17163=DIRECTION('ref_axis',(1.,0.,0.));
#17164=DIRECTION('center_axis',(1.,0.,0.));
#17165=DIRECTION('ref_axis',(0.,0.707106781186548,0.707106781186547));
#17166=DIRECTION('center_axis',(-1.,0.,0.));
#17167=DIRECTION('ref_axis',(0.,0.707106781186548,0.707106781186547));
#17168=DIRECTION('',(-1.,0.,0.));
#17169=DIRECTION('center_axis',(-1.,0.,0.));
#17170=DIRECTION('ref_axis',(0.,0.707106781186548,0.707106781186547));
#17171=DIRECTION('',(1.,0.,0.));
#17172=DIRECTION('center_axis',(0.,1.,0.));
#17173=DIRECTION('ref_axis',(0.,0.,1.));
#17174=DIRECTION('',(0.,0.,-1.));
#17175=DIRECTION('',(-0.707106781186547,0.,-0.707106781186547));
#17176=DIRECTION('',(-1.,0.,0.));
#17177=DIRECTION('',(0.,0.,-1.));
#17178=DIRECTION('center_axis',(0.,-1.,0.));
#17179=DIRECTION('ref_axis',(1.,0.,0.));
#17180=DIRECTION('center_axis',(0.,1.,0.));
#17181=DIRECTION('ref_axis',(1.,0.,0.));
#17182=DIRECTION('',(0.,1.,0.));
#17183=DIRECTION('center_axis',(0.,0.,-1.));
#17184=DIRECTION('ref_axis',(-1.,0.,0.));
#17185=DIRECTION('',(0.,1.,0.));
#17186=DIRECTION('center_axis',(0.707106781186548,0.,-0.707106781186548));
#17187=DIRECTION('ref_axis',(-0.707106781186548,0.,-0.707106781186548));
#17188=DIRECTION('',(0.,1.,0.));
#17189=DIRECTION('center_axis',(0.,0.,-1.));
#17190=DIRECTION('ref_axis',(-0.707106781186548,-0.707106781186548,0.));
#17191=DIRECTION('center_axis',(0.,0.,1.));
#17192=DIRECTION('ref_axis',(-0.707106781186548,-0.707106781186548,0.));
#17193=DIRECTION('',(0.,0.,1.));
#17194=DIRECTION('center_axis',(0.,0.,-1.));
#17195=DIRECTION('ref_axis',(-0.707106781186548,-0.707106781186548,0.));
#17196=DIRECTION('',(0.,0.,-1.));
#17197=DIRECTION('center_axis',(-1.,0.,0.));
#17198=DIRECTION('ref_axis',(0.,0.,-1.));
#17199=DIRECTION('',(0.,-1.,0.));
#17200=DIRECTION('',(0.,-1.,0.));
#17201=DIRECTION('center_axis',(-1.,0.,0.));
#17202=DIRECTION('ref_axis',(0.,0.,-1.));
#17203=DIRECTION('center_axis',(1.,0.,0.));
#17204=DIRECTION('ref_axis',(0.,-0.707106781186548,0.707106781186547));
#17205=DIRECTION('',(0.,-1.,0.));
#17206=DIRECTION('',(0.,1.,0.));
#17207=DIRECTION('center_axis',(-1.,0.,0.));
#17208=DIRECTION('ref_axis',(0.,-0.707106781186548,0.707106781186547));
#17209=DIRECTION('',(0.,0.,-1.));
#17210=DIRECTION('',(0.,-1.,0.));
#17211=DIRECTION('',(0.,0.,-1.));
#17212=DIRECTION('center_axis',(0.,-1.,0.));
#17213=DIRECTION('ref_axis',(-1.,0.,0.));
#17214=DIRECTION('center_axis',(0.,1.,0.));
#17215=DIRECTION('ref_axis',(-1.,0.,0.));
#17216=DIRECTION('',(0.,-1.,0.));
#17217=DIRECTION('center_axis',(0.,1.,0.));
#17218=DIRECTION('ref_axis',(-1.,0.,0.));
#17219=DIRECTION('center_axis',(-0.707106781186548,0.,-0.707106781186548));
#17220=DIRECTION('ref_axis',(0.707106781186548,0.,-0.707106781186548));
#17221=DIRECTION('',(0.707106781186547,0.,-0.707106781186547));
#17222=DIRECTION('',(0.,-1.,0.));
#17223=DIRECTION('',(0.707106781186547,0.,-0.707106781186547));
#17224=DIRECTION('center_axis',(0.,0.,1.));
#17225=DIRECTION('ref_axis',(0.707106781186548,-0.707106781186548,0.));
#17226=DIRECTION('center_axis',(0.,0.,-1.));
#17227=DIRECTION('ref_axis',(0.707106781186548,-0.707106781186548,0.));
#17228=DIRECTION('',(0.,0.,-1.));
#17229=DIRECTION('center_axis',(0.,0.,1.));
#17230=DIRECTION('ref_axis',(0.707106781186548,-0.707106781186548,0.));
#17231=DIRECTION('',(0.,0.,1.));
#17232=DIRECTION('center_axis',(0.,1.,0.));
#17233=DIRECTION('ref_axis',(0.,0.,1.));
#17234=DIRECTION('',(-1.,0.,0.));
#17235=DIRECTION('',(-1.,0.,0.));
#17236=DIRECTION('center_axis',(0.,0.,1.));
#17237=DIRECTION('ref_axis',(-1.,0.,0.));
#17238=DIRECTION('',(0.,1.,0.));
#17239=DIRECTION('',(1.,0.,0.));
#17240=DIRECTION('',(0.,1.,0.));
#17241=DIRECTION('center_axis',(-1.,0.,0.));
#17242=DIRECTION('ref_axis',(0.,0.,-1.));
#17243=DIRECTION('',(0.,1.,0.));
#17244=DIRECTION('center_axis',(0.,0.,-1.));
#17245=DIRECTION('ref_axis',(1.,0.,0.));
#17246=DIRECTION('center_axis',(-1.,0.,0.));
#17247=DIRECTION('ref_axis',(0.,-0.707106781186548,0.707106781186547));
#17248=DIRECTION('',(1.,0.,0.));
#17249=DIRECTION('',(-1.,0.,0.));
#17250=DIRECTION('center_axis',(-1.,0.,0.));
#17251=DIRECTION('ref_axis',(0.,-0.707106781186548,0.707106781186547));
#17252=DIRECTION('center_axis',(0.,-1.,0.));
#17253=DIRECTION('ref_axis',(1.,0.,0.));
#17254=DIRECTION('',(0.,0.,-1.));
#17255=DIRECTION('',(-0.707106781186547,0.,-0.707106781186547));
#17256=DIRECTION('',(1.,0.,0.));
#17257=DIRECTION('center_axis',(0.,-1.,0.));
#17258=DIRECTION('ref_axis',(1.,0.,0.));
#17259=DIRECTION('center_axis',(-1.,0.,0.));
#17260=DIRECTION('ref_axis',(0.,-0.707106781186548,0.707106781186547));
#17261=DIRECTION('center_axis',(1.,0.,0.));
#17262=DIRECTION('ref_axis',(0.,-0.707106781186548,0.707106781186547));
#17263=DIRECTION('',(-1.,0.,0.));
#17264=DIRECTION('center_axis',(0.,1.,0.));
#17265=DIRECTION('ref_axis',(0.,0.,1.));
#17266=DIRECTION('',(-1.,0.,0.));
#17267=DIRECTION('',(-0.707106781186547,0.,-0.707106781186547));
#17268=DIRECTION('',(0.,0.,-1.));
#17269=DIRECTION('center_axis',(0.,-1.,0.));
#17270=DIRECTION('ref_axis',(1.,0.,0.));
#17271=DIRECTION('center_axis',(-1.,0.,0.));
#17272=DIRECTION('ref_axis',(0.,0.,-1.));
#17273=DIRECTION('',(0.,-1.,0.));
#17274=DIRECTION('',(0.,1.,0.));
#17275=DIRECTION('center_axis',(0.,1.,0.));
#17276=DIRECTION('ref_axis',(1.,0.,0.));
#17277=DIRECTION('',(0.,1.,0.));
#17278=DIRECTION('center_axis',(0.,0.,1.));
#17279=DIRECTION('ref_axis',(-1.,0.,0.));
#17280=DIRECTION('',(0.,-1.,0.));
#17281=DIRECTION('center_axis',(-0.707106781186548,0.,0.707106781186548));
#17282=DIRECTION('ref_axis',(-0.707106781186548,0.,-0.707106781186548));
#17283=DIRECTION('center_axis',(0.,0.,1.));
#17284=DIRECTION('ref_axis',(-1.,0.,0.));
#240633=CARTESIAN_POINT('',(0.,0.,0.));
#240634=CARTESIAN_POINT('Origin',(-39.9751670169646,25.,260.358721235131));
#240635=CARTESIAN_POINT('',(-49.9751670169646,25.,256.608721235131));
#240636=CARTESIAN_POINT('',(-39.9751670169646,35.,256.608721235131));
#240637=CARTESIAN_POINT('Origin',(-39.9751670169646,25.,256.608721235131));
#240638=CARTESIAN_POINT('',(-49.9751670169646,25.,261.608721235131));
#240639=CARTESIAN_POINT('',(-49.9751670169646,25.,260.358721235131));
#240640=CARTESIAN_POINT('',(-39.9751670169646,35.,261.608721235131));
#240641=CARTESIAN_POINT('Origin',(-39.9751670169646,25.,261.608721235131));
#240642=CARTESIAN_POINT('',(-39.9751670169646,35.,260.358721235131));
#240643=CARTESIAN_POINT('Origin',(-19.9792411332937,0.,231.631408332131));
#240644=CARTESIAN_POINT('',(-12.4213924902778,25.,231.631408332131));
#240645=CARTESIAN_POINT('Origin',(-19.9792411332937,25.,231.631408332131));
#240646=CARTESIAN_POINT('',(-12.4213924902778,22.,231.631408332131));
#240647=CARTESIAN_POINT('',(-12.4213924902778,0.,231.631408332131));
#240648=CARTESIAN_POINT('Origin',(-19.9792411332937,22.,231.631408332131));
#240649=CARTESIAN_POINT('Origin',(-35.0075079285187,0.,224.577877459809));
#240650=CARTESIAN_POINT('',(-35.0075079285187,22.,224.577877459809));
#240651=CARTESIAN_POINT('',(-27.0075079285187,22.,216.577877459809));
#240652=CARTESIAN_POINT('',(-33.010424909369,22.,222.58079444066));
#240653=CARTESIAN_POINT('',(-35.0075079285187,25.,224.577877459809));
#240654=CARTESIAN_POINT('',(-35.0075079285187,0.,224.577877459809));
#240655=CARTESIAN_POINT('',(-27.0075079285187,25.,216.577877459809));
#240656=CARTESIAN_POINT('',(-35.0075079285187,25.,224.577877459809));
#240657=CARTESIAN_POINT('',(-27.0075079285187,0.,216.577877459809));
#240658=CARTESIAN_POINT('Origin',(39.9751670169646,25.,260.358721235131));
#240659=CARTESIAN_POINT('',(49.9751670169646,25.,256.608721235131));
#240660=CARTESIAN_POINT('',(39.9751670169646,35.,256.608721235131));
#240661=CARTESIAN_POINT('Origin',(39.9751670169646,25.,256.608721235131));
#240662=CARTESIAN_POINT('',(39.9751670169646,35.,261.608721235131));
#240663=CARTESIAN_POINT('',(39.9751670169646,35.,260.358721235131));
#240664=CARTESIAN_POINT('',(49.9751670169646,25.,261.608721235131));
#240665=CARTESIAN_POINT('Origin',(39.9751670169646,25.,261.608721235131));
#240666=CARTESIAN_POINT('',(49.9751670169646,25.,260.358721235131));
#240667=CARTESIAN_POINT('Origin',(24.9875835084823,35.,259.108721235131));
#240668=CARTESIAN_POINT('',(0.,35.,256.608721235131));
#240669=CARTESIAN_POINT('',(0.,35.,261.608721235131));
#240670=CARTESIAN_POINT('Origin',(26.255630946389,19.,248.608721235131));
#240671=CARTESIAN_POINT('',(-35.0075079285187,22.,248.608721235131));
#240672=CARTESIAN_POINT('',(35.0075079285187,22.,248.608721235131));
#240673=CARTESIAN_POINT('',(26.255630946389,22.,248.608721235131));
#240674=CARTESIAN_POINT('',(35.0075079285187,19.,251.608721235131));
#240675=CARTESIAN_POINT('Origin',(35.0075079285187,19.,248.608721235131));
#240676=CARTESIAN_POINT('',(-35.0075079285187,19.,251.608721235131));
#240677=CARTESIAN_POINT('',(26.255630946389,19.,251.608721235131));
#240678=CARTESIAN_POINT('Origin',(-35.0075079285187,19.,248.608721235131));
#240679=CARTESIAN_POINT('Origin',(17.5037539642593,22.,234.09329934747));
#240680=CARTESIAN_POINT('',(-35.0075079285187,22.,242.851010291301));
#240681=CARTESIAN_POINT('',(27.0075079285187,22.,216.577877459809));
#240682=CARTESIAN_POINT('',(-22.255630946389,22.,216.577877459809));
#240683=CARTESIAN_POINT('',(35.0075079285187,22.,224.577877459809));
#240684=CARTESIAN_POINT('',(33.010424909369,22.,222.58079444066));
#240685=CARTESIAN_POINT('',(35.0075079285187,22.,242.851010291301));
#240686=CARTESIAN_POINT('',(12.4213924902778,22.,231.631408332131));
#240687=CARTESIAN_POINT('Origin',(19.9792411332937,22.,231.631408332131));
#240688=CARTESIAN_POINT('Origin',(8.75187698212967,19.5,251.108721235131));
#240689=CARTESIAN_POINT('',(35.0075079285187,19.5,256.608721235131));
#240690=CARTESIAN_POINT('',(35.0075079285187,25.,251.108721235131));
#240691=CARTESIAN_POINT('Origin',(35.0075079285187,19.5,251.108721235131));
#240692=CARTESIAN_POINT('',(-35.0075079285187,25.,251.108721235131));
#240693=CARTESIAN_POINT('',(8.75187698212967,25.,251.108721235131));
#240694=CARTESIAN_POINT('',(-35.0075079285187,19.5,256.608721235131));
#240695=CARTESIAN_POINT('Origin',(-35.0075079285187,19.5,251.108721235131));
#240696=CARTESIAN_POINT('',(8.75187698212967,19.5,256.608721235131));
#240697=CARTESIAN_POINT('Origin',(17.5037539642593,25.,254.108721235131));
#240698=CARTESIAN_POINT('',(35.0075079285187,25.,224.577877459809));
#240699=CARTESIAN_POINT('',(35.0075079285187,25.,256.608721235131));
#240700=CARTESIAN_POINT('',(27.0075079285187,25.,216.577877459809));
#240701=CARTESIAN_POINT('',(35.0075079285187,25.,224.577877459809));
#240702=CARTESIAN_POINT('',(27.0075079285187,25.,216.577877459809));
#240703=CARTESIAN_POINT('',(-35.0075079285187,25.,256.608721235131));
#240704=CARTESIAN_POINT('',(12.4213924902778,25.,231.631408332131));
#240705=CARTESIAN_POINT('Origin',(19.9792411332937,25.,231.631408332131));
#240706=CARTESIAN_POINT('Origin',(19.9792411332937,0.,231.631408332131));
#240707=CARTESIAN_POINT('',(12.4213924902778,0.,231.631408332131));
#240708=CARTESIAN_POINT('Origin',(27.0075079285187,0.,216.577877459809));
#240709=CARTESIAN_POINT('',(27.0075079285187,0.,216.577877459809));
#240710=CARTESIAN_POINT('Origin',(35.0075079285187,0.,224.577877459809));
#240711=CARTESIAN_POINT('',(35.0075079285187,0.,224.577877459809));
#240712=CARTESIAN_POINT('Origin',(-39.9751670169646,-25.,260.358721235131));
#240713=CARTESIAN_POINT('',(-49.9751670169646,-25.,256.608721235131));
#240714=CARTESIAN_POINT('',(-39.9751670169646,-35.,256.608721235131));
#240715=CARTESIAN_POINT('Origin',(-39.9751670169646,-25.,256.608721235131));
#240716=CARTESIAN_POINT('',(-39.9751670169646,-35.,261.608721235131));
#240717=CARTESIAN_POINT('',(-39.9751670169646,-35.,260.358721235131));
#240718=CARTESIAN_POINT('',(-49.9751670169646,-25.,261.608721235131));
#240719=CARTESIAN_POINT('Origin',(-39.9751670169646,-25.,261.608721235131));
#240720=CARTESIAN_POINT('',(-49.9751670169646,-25.,260.358721235131));
#240721=CARTESIAN_POINT('Origin',(-49.9751670169646,0.,261.608721235131));
#240722=CARTESIAN_POINT('',(-49.9751670169646,0.,261.608721235131));
#240723=CARTESIAN_POINT('',(-49.9751670169646,0.,256.608721235131));
#240724=CARTESIAN_POINT('Origin',(-35.0075079285187,0.,256.608721235131));
#240725=CARTESIAN_POINT('',(-35.0075079285187,-19.5,256.608721235131));
#240726=CARTESIAN_POINT('',(-35.0075079285187,-25.,251.108721235131));
#240727=CARTESIAN_POINT('Origin',(-35.0075079285187,-19.5,251.108721235131));
#240728=CARTESIAN_POINT('',(-35.0075079285187,0.,256.608721235131));
#240729=CARTESIAN_POINT('',(-35.0075079285187,-19.,251.608721235131));
#240730=CARTESIAN_POINT('',(-35.0075079285187,0.,251.608721235131));
#240731=CARTESIAN_POINT('',(-35.0075079285187,-22.,248.608721235131));
#240732=CARTESIAN_POINT('Origin',(-35.0075079285187,-19.,248.608721235131));
#240733=CARTESIAN_POINT('',(-35.0075079285187,-22.,224.577877459809));
#240734=CARTESIAN_POINT('',(-35.0075079285187,-22.,242.851010291301));
#240735=CARTESIAN_POINT('',(-35.0075079285187,-25.,224.577877459809));
#240736=CARTESIAN_POINT('',(-35.0075079285187,0.,224.577877459809));
#240737=CARTESIAN_POINT('',(-35.0075079285187,-25.,256.608721235131));
#240738=CARTESIAN_POINT('Origin',(-19.9792411332937,0.,231.631408332131));
#240739=CARTESIAN_POINT('',(-12.4213924902778,-22.,231.631408332131));
#240740=CARTESIAN_POINT('Origin',(-19.9792411332937,-22.,231.631408332131));
#240741=CARTESIAN_POINT('',(-12.4213924902778,-25.,231.631408332131));
#240742=CARTESIAN_POINT('',(-12.4213924902778,0.,231.631408332131));
#240743=CARTESIAN_POINT('Origin',(-19.9792411332937,-25.,231.631408332131));
#240744=CARTESIAN_POINT('Origin',(-35.0075079285187,0.,224.577877459809));
#240745=CARTESIAN_POINT('',(-27.0075079285187,-22.,216.577877459809));
#240746=CARTESIAN_POINT('',(-33.010424909369,-22.,222.58079444066));
#240747=CARTESIAN_POINT('',(-27.0075079285187,-25.,216.577877459809));
#240748=CARTESIAN_POINT('',(-27.0075079285187,0.,216.577877459809));
#240749=CARTESIAN_POINT('',(-35.0075079285187,-25.,224.577877459809));
#240750=CARTESIAN_POINT('Origin',(39.9751670169646,-25.,260.358721235131));
#240751=CARTESIAN_POINT('',(49.9751670169646,-25.,256.608721235131));
#240752=CARTESIAN_POINT('',(39.9751670169646,-35.,256.608721235131));
#240753=CARTESIAN_POINT('Origin',(39.9751670169646,-25.,256.608721235131));
#240754=CARTESIAN_POINT('',(49.9751670169646,-25.,261.608721235131));
#240755=CARTESIAN_POINT('',(49.9751670169646,-25.,260.358721235131));
#240756=CARTESIAN_POINT('',(39.9751670169646,-35.,261.608721235131));
#240757=CARTESIAN_POINT('Origin',(39.9751670169646,-25.,261.608721235131));
#240758=CARTESIAN_POINT('',(39.9751670169646,-35.,260.358721235131));
#240759=CARTESIAN_POINT('Origin',(24.9875835084823,-35.,259.108721235131));
#240760=CARTESIAN_POINT('',(0.,-35.,261.608721235131));
#240761=CARTESIAN_POINT('',(0.,-35.,256.608721235131));
#240762=CARTESIAN_POINT('Origin',(49.9751670169646,0.,256.608721235131));
#240763=CARTESIAN_POINT('',(49.9751670169646,0.,256.608721235131));
#240764=CARTESIAN_POINT('',(35.0075079285187,-19.5,256.608721235131));
#240765=CARTESIAN_POINT('',(8.75187698212967,-19.5,256.608721235131));
#240766=CARTESIAN_POINT('',(35.0075079285187,0.,256.608721235131));
#240767=CARTESIAN_POINT('Origin',(49.9751670169646,0.,261.608721235131));
#240768=CARTESIAN_POINT('',(49.9751670169646,0.,261.608721235131));
#240769=CARTESIAN_POINT('Origin',(0.,0.,261.608721235131));
#240770=CARTESIAN_POINT('Origin',(26.255630946389,-19.,248.608721235131));
#240771=CARTESIAN_POINT('',(35.0075079285187,-22.,248.608721235131));
#240772=CARTESIAN_POINT('',(26.255630946389,-22.,248.608721235131));
#240773=CARTESIAN_POINT('',(35.0075079285187,-19.,251.608721235131));
#240774=CARTESIAN_POINT('',(26.255630946389,-19.,251.608721235131));
#240775=CARTESIAN_POINT('Origin',(35.0075079285187,-19.,248.608721235131));
#240776=CARTESIAN_POINT('Origin',(17.5037539642593,-22.,234.09329934747));
#240777=CARTESIAN_POINT('',(35.0075079285187,-22.,224.577877459809));
#240778=CARTESIAN_POINT('',(35.0075079285187,-22.,242.851010291301));
#240779=CARTESIAN_POINT('',(27.0075079285187,-22.,216.577877459809));
#240780=CARTESIAN_POINT('',(33.010424909369,-22.,222.58079444066));
#240781=CARTESIAN_POINT('',(-22.255630946389,-22.,216.577877459809));
#240782=CARTESIAN_POINT('',(12.4213924902778,-22.,231.631408332131));
#240783=CARTESIAN_POINT('Origin',(19.9792411332937,-22.,231.631408332131));
#240784=CARTESIAN_POINT('Origin',(8.75187698212967,-19.5,251.108721235131));
#240785=CARTESIAN_POINT('',(35.0075079285187,-25.,251.108721235131));
#240786=CARTESIAN_POINT('Origin',(35.0075079285187,-19.5,251.108721235131));
#240787=CARTESIAN_POINT('',(8.75187698212967,-25.,251.108721235131));
#240788=CARTESIAN_POINT('Origin',(17.5037539642593,-25.,254.108721235131));
#240789=CARTESIAN_POINT('',(27.0075079285187,-25.,216.577877459809));
#240790=CARTESIAN_POINT('',(27.0075079285187,-25.,216.577877459809));
#240791=CARTESIAN_POINT('',(35.0075079285187,-25.,224.577877459809));
#240792=CARTESIAN_POINT('',(35.0075079285187,-25.,224.577877459809));
#240793=CARTESIAN_POINT('',(35.0075079285187,-25.,256.608721235131));
#240794=CARTESIAN_POINT('',(12.4213924902778,-25.,231.631408332131));
#240795=CARTESIAN_POINT('Origin',(19.9792411332937,-25.,231.631408332131));
#240796=CARTESIAN_POINT('Origin',(35.0075079285187,0.,256.608721235131));
#240797=CARTESIAN_POINT('',(35.0075079285187,0.,224.577877459809));
#240798=CARTESIAN_POINT('',(35.0075079285187,0.,251.608721235131));
#240799=CARTESIAN_POINT('Origin',(19.9792411332937,0.,231.631408332131));
#240800=CARTESIAN_POINT('',(12.4213924902778,0.,231.631408332131));
#240801=CARTESIAN_POINT('Origin',(27.0075079285187,0.,216.577877459809));
#240802=CARTESIAN_POINT('',(27.0075079285187,0.,216.577877459809));
#240803=CARTESIAN_POINT('Origin',(35.0075079285187,0.,224.577877459809));
#240804=CARTESIAN_POINT('Origin',(35.0075079285187,0.,251.608721235131));
#279252=UNCERTAINTY_MEASURE_WITH_UNIT(LENGTH_MEASURE(0.01),#279267,
'DISTANCE_ACCURACY_VALUE',
'Maximum model space distance between geometric entities at asserted c
onnectivities');
#279255=UNCERTAINTY_MEASURE_WITH_UNIT(LENGTH_MEASURE(0.01),#279267,
'DISTANCE_ACCURACY_VALUE',
'Maximum model space distance between geometric entities at asserted c
onnectivities');
#279263=(
GEOMETRIC_REPRESENTATION_CONTEXT(3)
GLOBAL_UNCERTAINTY_ASSIGNED_CONTEXT((#279252))
GLOBAL_UNIT_ASSIGNED_CONTEXT((#279267,#279269,#279270))
REPRESENTATION_CONTEXT('','3D')
);
#279266=(
GEOMETRIC_REPRESENTATION_CONTEXT(3)
GLOBAL_UNCERTAINTY_ASSIGNED_CONTEXT((#279255))
GLOBAL_UNIT_ASSIGNED_CONTEXT((#279267,#279269,#279270))
REPRESENTATION_CONTEXT('','3D')
);
#279267=(
LENGTH_UNIT()
NAMED_UNIT(*)
SI_UNIT(.MILLI.,.METRE.)
);
#279269=(
NAMED_UNIT(*)
PLANE_ANGLE_UNIT()
SI_UNIT($,.RADIAN.)
);
#279270=(
NAMED_UNIT(*)
SI_UNIT($,.STERADIAN.)
SOLID_ANGLE_UNIT()
);
#279278=SHAPE_DEFINITION_REPRESENTATION(#279288,#279307);
#279288=PRODUCT_DEFINITION_SHAPE('',$,#279318);
#279307=SHAPE_REPRESENTATION('',(#15552),#279263);
#279310=PRODUCT_DEFINITION_CONTEXT('part definition',#279342,'design');
#279318=PRODUCT_DEFINITION('Top_Part','Top_Part',#279328,#279310);
#279328=PRODUCT_DEFINITION_FORMATION('',$,#279351);
#279342=APPLICATION_CONTEXT(
'Core Data for Automotive Mechanical Design Process');
#279343=PRODUCT_CONTEXT('part definition',#279342,'mechanical');
#279351=PRODUCT('Top_Part','Top_Part',$,(#279343));
#279355=PRESENTATION_STYLE_ASSIGNMENT((#279357));
#279357=SURFACE_STYLE_USAGE(.BOTH.,#279359);
#279359=SURFACE_SIDE_STYLE('',(#279361));
#279361=SURFACE_STYLE_FILL_AREA(#279363);
#279363=FILL_AREA_STYLE('Opaque(160,160,160)',(#279365));
#279365=FILL_AREA_STYLE_COLOUR('Opaque(160,160,160)',#279367);
#279367=COLOUR_RGB('Opaque(160,160,160)', 0.66274510, 0.83137255, 0.94901961);
ENDSEC;
END-ISO-10303-21;
